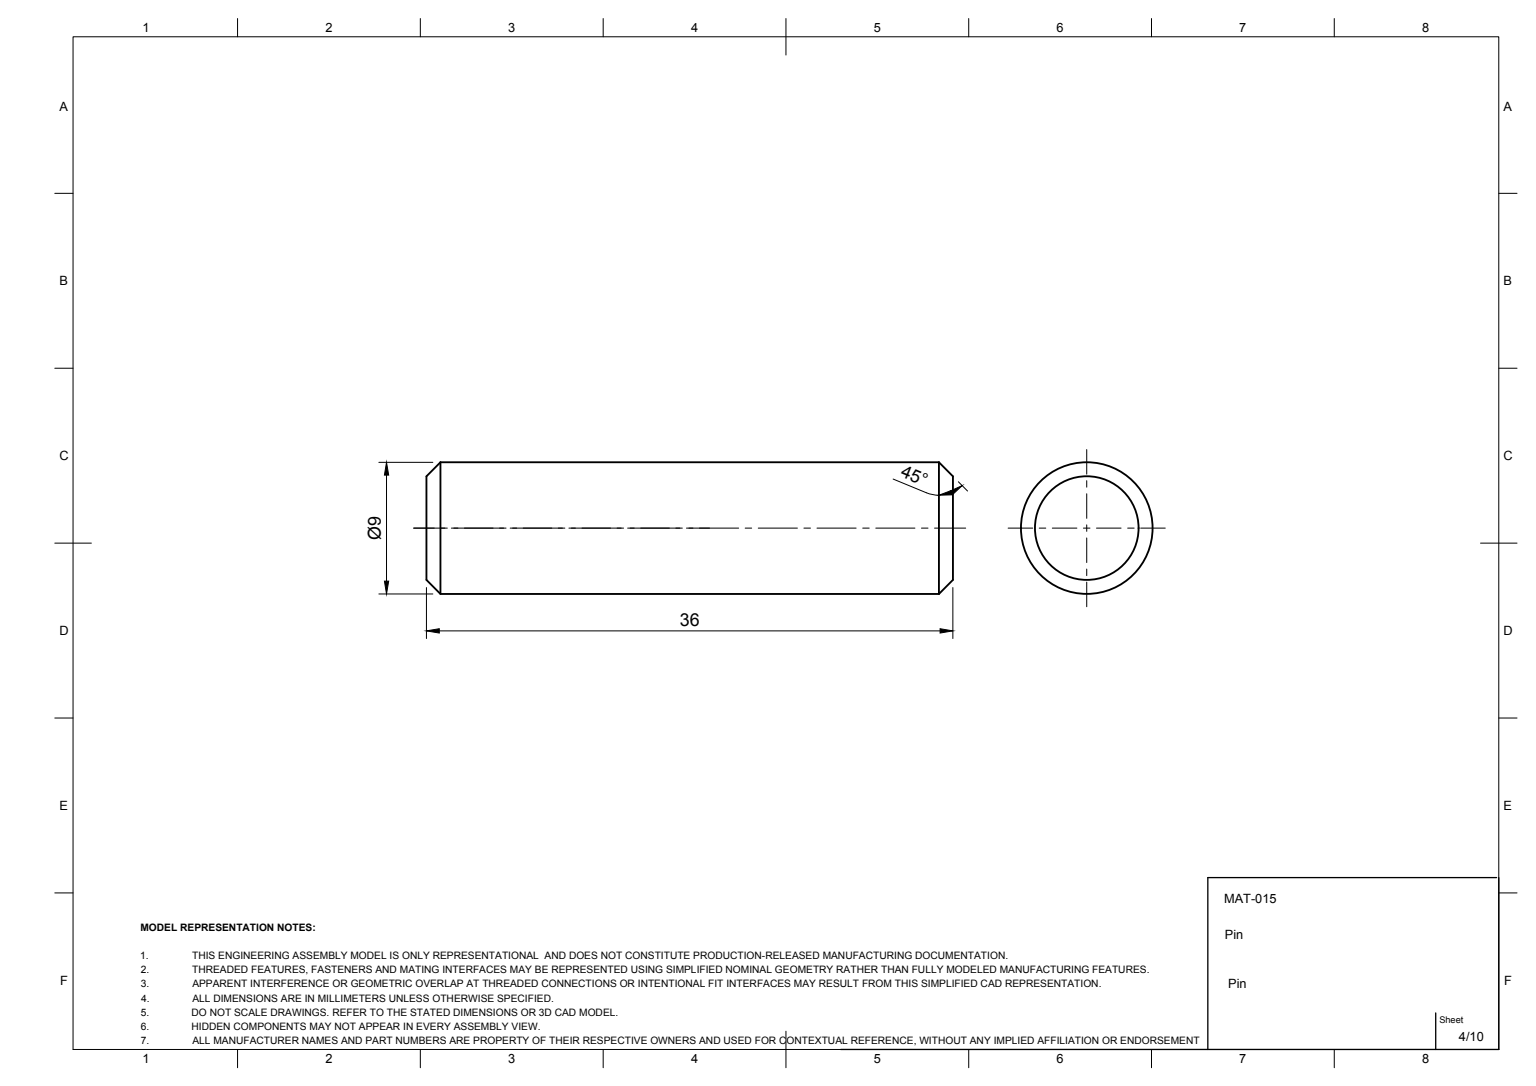
ISO-10303-21;
HEADER;
/* Generated by software containing ST-Developer
 * from STEP Tools, Inc. (www.steptools.com) 
 */

FILE_DESCRIPTION(
/* description */ ('STEP AP214'),
/* implementation_level */ '2;1');

FILE_NAME(
/* name */ 'Pin.step',
/* time_stamp */ '2026-11-14T06:03:18-08:00',
/* author */ (''),
/* organization */ (''),
/* preprocessor_version */ 'ST-DEVELOPER v20.2',
/* originating_system */ 'Autodesk Translation Framework v15.17.0.0',
/* authorisation */ '');

FILE_SCHEMA (('AUTOMOTIVE_DESIGN { 1 0 10303 214 3 1 1 }'));
ENDSEC;

DATA;
#10=MECHANICAL_DESIGN_GEOMETRIC_PRESENTATION_REPRESENTATION('',(#79),#3206);
#54=CONICAL_SURFACE('',#2056,4.50000000000002,0.785398163397454);
#55=CONICAL_SURFACE('',#2059,3.54000000000001,0.785398163397446);
#63=SHAPE_REPRESENTATION_RELATIONSHIP('SRR','None',#3246,#71);
#71=ADVANCED_BREP_SHAPE_REPRESENTATION('',(#87),#3205);
#79=STYLED_ITEM('',(#3290),#87);
#87=MANIFOLD_SOLID_BREP('Body1',#1786);
#145=PLANE('',#2064);
#146=PLANE('',#2065);
#330=LINE('',#3164,#475);
#331=LINE('',#3172,#476);
#332=LINE('',#3175,#477);
#475=VECTOR('',#2581,4.50000000000002);
#476=VECTOR('',#2590,3.54000000000001);
#477=VECTOR('',#2595,4.50000000000002);
#511=CYLINDRICAL_SURFACE('',#2063,4.50000000000002);
#607=FACE_OUTER_BOUND('',#748,.T.);
#608=FACE_OUTER_BOUND('',#749,.T.);
#609=FACE_OUTER_BOUND('',#750,.T.);
#610=FACE_OUTER_BOUND('',#751,.T.);
#611=FACE_OUTER_BOUND('',#752,.T.);
#748=EDGE_LOOP('',(#1661,#1662,#1663,#1664));
#749=EDGE_LOOP('',(#1665,#1666,#1667,#1668,#1669));
#750=EDGE_LOOP('',(#1670,#1671,#1672,#1673,#1674));
#751=EDGE_LOOP('',(#1675));
#752=EDGE_LOOP('',(#1676));
#829=CIRCLE('',#2057,4.50000000000002);
#830=CIRCLE('',#2058,3.54);
#831=CIRCLE('',#2060,4.50000000000002);
#832=CIRCLE('',#2061,4.50000000000002);
#833=CIRCLE('',#2062,3.54000000000001);
#982=VERTEX_POINT('',#3161);
#983=VERTEX_POINT('',#3163);
#984=VERTEX_POINT('',#3167);
#985=VERTEX_POINT('',#3168);
#986=VERTEX_POINT('',#3171);
#1209=EDGE_CURVE('',#982,#982,#829,.T.);
#1210=EDGE_CURVE('',#982,#983,#330,.T.);
#1211=EDGE_CURVE('',#983,#983,#830,.T.);
#1212=EDGE_CURVE('',#984,#985,#831,.T.);
#1213=EDGE_CURVE('',#985,#984,#832,.T.);
#1214=EDGE_CURVE('',#985,#986,#331,.T.);
#1215=EDGE_CURVE('',#986,#986,#833,.T.);
#1216=EDGE_CURVE('',#984,#982,#332,.T.);
#1661=ORIENTED_EDGE('',*,*,#1209,.F.);
#1662=ORIENTED_EDGE('',*,*,#1210,.T.);
#1663=ORIENTED_EDGE('',*,*,#1211,.F.);
#1664=ORIENTED_EDGE('',*,*,#1210,.F.);
#1665=ORIENTED_EDGE('',*,*,#1212,.F.);
#1666=ORIENTED_EDGE('',*,*,#1213,.F.);
#1667=ORIENTED_EDGE('',*,*,#1214,.T.);
#1668=ORIENTED_EDGE('',*,*,#1215,.F.);
#1669=ORIENTED_EDGE('',*,*,#1214,.F.);
#1670=ORIENTED_EDGE('',*,*,#1212,.T.);
#1671=ORIENTED_EDGE('',*,*,#1213,.T.);
#1672=ORIENTED_EDGE('',*,*,#1216,.T.);
#1673=ORIENTED_EDGE('',*,*,#1209,.T.);
#1674=ORIENTED_EDGE('',*,*,#1216,.F.);
#1675=ORIENTED_EDGE('',*,*,#1215,.T.);
#1676=ORIENTED_EDGE('',*,*,#1211,.T.);
#1774=ADVANCED_FACE('',(#607),#54,.T.);
#1775=ADVANCED_FACE('',(#608),#55,.T.);
#1776=ADVANCED_FACE('',(#609),#511,.T.);
#1777=ADVANCED_FACE('',(#610),#145,.T.);
#1778=ADVANCED_FACE('',(#611),#146,.T.);
#1786=CLOSED_SHELL('',(#1774,#1775,#1776,#1777,#1778));
#2055=AXIS2_PLACEMENT_3D('',#3159,#2575,#2576);
#2056=AXIS2_PLACEMENT_3D('',#3160,#2577,#2578);
#2057=AXIS2_PLACEMENT_3D('',#3162,#2579,#2580);
#2058=AXIS2_PLACEMENT_3D('',#3165,#2582,#2583);
#2059=AXIS2_PLACEMENT_3D('',#3166,#2584,#2585);
#2060=AXIS2_PLACEMENT_3D('',#3169,#2586,#2587);
#2061=AXIS2_PLACEMENT_3D('',#3170,#2588,#2589);
#2062=AXIS2_PLACEMENT_3D('',#3173,#2591,#2592);
#2063=AXIS2_PLACEMENT_3D('',#3174,#2593,#2594);
#2064=AXIS2_PLACEMENT_3D('',#3176,#2596,#2597);
#2065=AXIS2_PLACEMENT_3D('',#3177,#2598,#2599);
#2575=DIRECTION('axis',(0.,0.,1.));
#2576=DIRECTION('refdir',(1.,0.,0.));
#2577=DIRECTION('center_axis',(1.72563323017096E-31,-1.,-1.35585468084861E-31));
#2578=DIRECTION('ref_axis',(-5.55111512312577E-17,1.35585468084861E-31,
-1.));
#2579=DIRECTION('center_axis',(1.72563323017096E-31,-1.,-1.35585468084861E-31));
#2580=DIRECTION('ref_axis',(-8.32667268468868E-16,-1.35585468084862E-31,
1.));
#2581=DIRECTION('',(4.73432941564552E-17,0.707106781186544,-0.707106781186551));
#2582=DIRECTION('center_axis',(-1.72563323017096E-31,1.,1.35585468084861E-31));
#2583=DIRECTION('ref_axis',(5.55111512312576E-17,-1.35585468084861E-31,
1.));
#2584=DIRECTION('center_axis',(-1.72563323017096E-31,1.,1.35585468084861E-31));
#2585=DIRECTION('ref_axis',(5.55111512312576E-17,-1.35585468084861E-31,
1.));
#2586=DIRECTION('center_axis',(-1.72563323017096E-31,1.,1.35585468084861E-31));
#2587=DIRECTION('ref_axis',(-5.55111512312576E-17,1.35585468084861E-31,
-1.));
#2588=DIRECTION('center_axis',(-1.72563323017096E-31,1.,1.35585468084861E-31));
#2589=DIRECTION('ref_axis',(-5.55111512312576E-17,1.35585468084861E-31,
-1.));
#2590=DIRECTION('',(1.25847917090643E-16,-0.707106781186549,0.707106781186546));
#2591=DIRECTION('center_axis',(1.72563323017096E-31,-1.,-1.35585468084861E-31));
#2592=DIRECTION('ref_axis',(-5.55111512312576E-17,1.35585468084861E-31,
-1.));
#2593=DIRECTION('center_axis',(1.72563323017096E-31,-1.,-1.35585468084861E-31));
#2594=DIRECTION('ref_axis',(-5.55111512312576E-17,1.35585468084861E-31,
-1.));
#2595=DIRECTION('',(-1.72563323017096E-31,1.,1.35585468084861E-31));
#2596=DIRECTION('center_axis',(1.72563323017096E-31,-1.,1.10933564796704E-31));
#2597=DIRECTION('ref_axis',(-5.55111512312576E-17,-1.10933564796704E-31,
-1.));
#2598=DIRECTION('center_axis',(-1.72563323017096E-31,1.,-1.10933564796704E-31));
#2599=DIRECTION('ref_axis',(5.55111512312576E-17,1.10933564796704E-31,1.));
#3159=CARTESIAN_POINT('',(0.,0.,0.));
#3160=CARTESIAN_POINT('Origin',(-3.46944695195361E-15,29.04,1.38777878078145E-14));
#3161=CARTESIAN_POINT('',(-3.77073783102926E-15,29.04,4.50000000000003));
#3162=CARTESIAN_POINT('Origin',(-3.46944695195361E-15,29.04,1.38777878078145E-14));
#3163=CARTESIAN_POINT('',(-3.70646244349312E-15,30.,3.54000000000001));
#3164=CARTESIAN_POINT('',(-3.77073783102926E-15,29.04,4.50000000000003));
#3165=CARTESIAN_POINT('Origin',(-3.46944695195361E-15,30.,1.38777878078145E-14));
#3166=CARTESIAN_POINT('Origin',(0.,-5.99999999999999,0.));
#3167=CARTESIAN_POINT('',(8.00891240156965E-16,-5.03999999999999,4.5));
#3168=CARTESIAN_POINT('',(-8.00891240156971E-16,-5.03999999999998,-4.50000000000001));
#3169=CARTESIAN_POINT('Origin',(0.,-5.03999999999999,0.));
#3170=CARTESIAN_POINT('Origin',(0.,-5.03999999999999,0.));
#3171=CARTESIAN_POINT('',(-6.30034442256817E-16,-5.99999999999999,-3.54000000000001));
#3172=CARTESIAN_POINT('',(-6.30034442256817E-16,-5.99999999999999,-3.54000000000001));
#3173=CARTESIAN_POINT('Origin',(0.,-5.99999999999999,0.));
#3174=CARTESIAN_POINT('Origin',(0.,-5.99999999999999,0.));
#3175=CARTESIAN_POINT('',(-3.01290879075651E-16,-5.99999999999999,4.50000000000002));
#3176=CARTESIAN_POINT('Origin',(4.50000000000004,-5.99999999999999,2.08166817117217E-14));
#3177=CARTESIAN_POINT('Origin',(-3.46944695195361E-15,30.,1.38777878078145E-14));
#3195=UNCERTAINTY_MEASURE_WITH_UNIT(LENGTH_MEASURE(0.01),#3207,
'DISTANCE_ACCURACY_VALUE',
'Maximum model space distance between geometric entities at asserted c
onnectivities');
#3196=UNCERTAINTY_MEASURE_WITH_UNIT(LENGTH_MEASURE(0.01),#3207,
'DISTANCE_ACCURACY_VALUE',
'Maximum model space distance between geometric entities at asserted c
onnectivities');
#3205=(
GEOMETRIC_REPRESENTATION_CONTEXT(3)
GLOBAL_UNCERTAINTY_ASSIGNED_CONTEXT((#3195))
GLOBAL_UNIT_ASSIGNED_CONTEXT((#3207,#3209,#3210))
REPRESENTATION_CONTEXT('','3D')
);
#3206=(
GEOMETRIC_REPRESENTATION_CONTEXT(3)
GLOBAL_UNCERTAINTY_ASSIGNED_CONTEXT((#3196))
GLOBAL_UNIT_ASSIGNED_CONTEXT((#3207,#3209,#3210))
REPRESENTATION_CONTEXT('','3D')
);
#3207=(
LENGTH_UNIT()
NAMED_UNIT(*)
SI_UNIT(.MILLI.,.METRE.)
);
#3209=(
NAMED_UNIT(*)
PLANE_ANGLE_UNIT()
SI_UNIT($,.RADIAN.)
);
#3210=(
NAMED_UNIT(*)
SI_UNIT($,.STERADIAN.)
SOLID_ANGLE_UNIT()
);
#3219=SHAPE_DEFINITION_REPRESENTATION(#3228,#3246);
#3228=PRODUCT_DEFINITION_SHAPE('',$,#3256);
#3246=SHAPE_REPRESENTATION('',(#2055),#3205);
#3247=PRODUCT_DEFINITION_CONTEXT('part definition',#3276,'design');
#3256=PRODUCT_DEFINITION('Pin','Pin',#3265,#3247);
#3265=PRODUCT_DEFINITION_FORMATION('',$,#3286);
#3276=APPLICATION_CONTEXT(
'Core Data for Automotive Mechanical Design Process');
#3277=PRODUCT_CONTEXT('part definition',#3276,'mechanical');
#3286=PRODUCT('Pin','Pin',$,(#3277));
#3290=PRESENTATION_STYLE_ASSIGNMENT((#3294));
#3294=SURFACE_STYLE_USAGE(.BOTH.,#3298);
#3298=SURFACE_SIDE_STYLE('',(#3302));
#3302=SURFACE_STYLE_FILL_AREA(#3306);
#3306=FILL_AREA_STYLE('Opaque(227,224,212)',(#3310));
#3310=FILL_AREA_STYLE_COLOUR('Opaque(227,224,212)',#3314);
#3314=COLOUR_RGB('Opaque(227,224,212)',0.890196078431372,0.87843137254902,
0.831372549019608);
ENDSEC;
END-ISO-10303-21;
